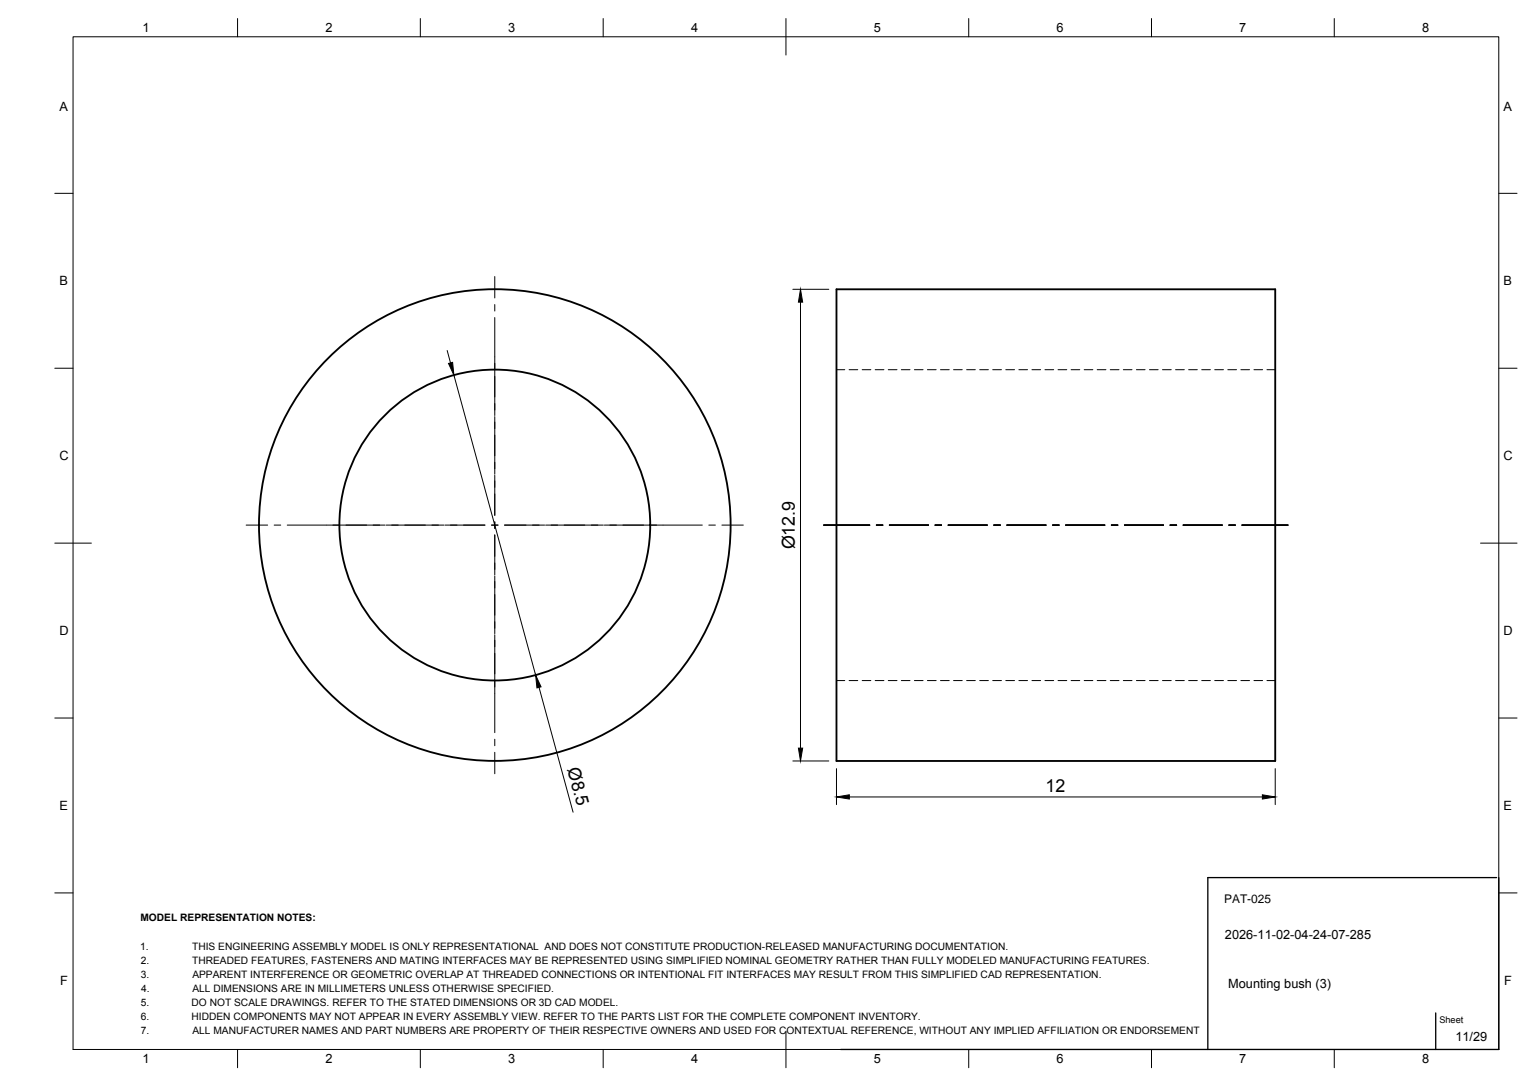
ISO-10303-21;
HEADER;
/* Generated by software containing ST-Developer
 * from STEP Tools, Inc. (www.steptools.com) 
 */

FILE_DESCRIPTION(
/* description */ ('Counter shaft with two pulleys and keyed hub'),
/* implementation_level */ '2;1');

FILE_NAME(
/* name */ 'Mounting bush (3).step',
/* time_stamp */ '2026-10-27T10:46:10-07:00',
/* author */ (''),
/* organization */ (''),
/* preprocessor_version */ 'ST-DEVELOPER v20.2',
/* originating_system */ 'Autodesk Translation Framework v15.17.0.0',
/* authorisation */ '');

FILE_SCHEMA (('AUTOMOTIVE_DESIGN { 1 0 10303 214 3 1 1 }'));
ENDSEC;

DATA;
#10=MECHANICAL_DESIGN_GEOMETRIC_PRESENTATION_REPRESENTATION('',(#296),#10821);
#246=SHAPE_REPRESENTATION_RELATIONSHIP('SRR','None',#10932,#271);
#271=ADVANCED_BREP_SHAPE_REPRESENTATION('',(#322),#10800);
#296=STYLED_ITEM('',(#11128),#322);
#322=MANIFOLD_SOLID_BREP('Body1',#5579);
#354=FACE_BOUND('',#953,.T.);
#355=FACE_BOUND('',#955,.T.);
#455=PLANE('',#5946);
#456=PLANE('',#5947);
#622=FACE_OUTER_BOUND('',#950,.T.);
#623=FACE_OUTER_BOUND('',#951,.T.);
#624=FACE_OUTER_BOUND('',#952,.T.);
#625=FACE_OUTER_BOUND('',#954,.T.);
#950=EDGE_LOOP('',(#3761,#3762,#3763,#3764));
#951=EDGE_LOOP('',(#3765,#3766,#3767,#3768));
#952=EDGE_LOOP('',(#3769));
#953=EDGE_LOOP('',(#3770));
#954=EDGE_LOOP('',(#3771));
#955=EDGE_LOOP('',(#3772));
#1353=LINE('',#8469,#1742);
#1354=LINE('',#8475,#1743);
#1742=VECTOR('',#6735,0.425);
#1743=VECTOR('',#6742,0.645);
#2105=CIRCLE('',#5941,0.425);
#2106=CIRCLE('',#5942,0.425);
#2107=CIRCLE('',#5944,0.645);
#2108=CIRCLE('',#5945,0.645);
#2428=VERTEX_POINT('',#8466);
#2429=VERTEX_POINT('',#8468);
#2430=VERTEX_POINT('',#8472);
#2431=VERTEX_POINT('',#8474);
#2953=EDGE_CURVE('',#2428,#2428,#2105,.T.);
#2954=EDGE_CURVE('',#2428,#2429,#1353,.T.);
#2955=EDGE_CURVE('',#2429,#2429,#2106,.T.);
#2956=EDGE_CURVE('',#2430,#2430,#2107,.T.);
#2957=EDGE_CURVE('',#2430,#2431,#1354,.T.);
#2958=EDGE_CURVE('',#2431,#2431,#2108,.T.);
#3761=ORIENTED_EDGE('',*,*,#2953,.F.);
#3762=ORIENTED_EDGE('',*,*,#2954,.T.);
#3763=ORIENTED_EDGE('',*,*,#2955,.T.);
#3764=ORIENTED_EDGE('',*,*,#2954,.F.);
#3765=ORIENTED_EDGE('',*,*,#2956,.F.);
#3766=ORIENTED_EDGE('',*,*,#2957,.T.);
#3767=ORIENTED_EDGE('',*,*,#2958,.T.);
#3768=ORIENTED_EDGE('',*,*,#2957,.F.);
#3769=ORIENTED_EDGE('',*,*,#2956,.T.);
#3770=ORIENTED_EDGE('',*,*,#2953,.T.);
#3771=ORIENTED_EDGE('',*,*,#2958,.F.);
#3772=ORIENTED_EDGE('',*,*,#2955,.F.);
#5123=CYLINDRICAL_SURFACE('',#5940,0.425);
#5124=CYLINDRICAL_SURFACE('',#5943,0.645);
#5293=ADVANCED_FACE('',(#622),#5123,.F.);
#5294=ADVANCED_FACE('',(#623),#5124,.T.);
#5295=ADVANCED_FACE('',(#624,#354),#455,.T.);
#5296=ADVANCED_FACE('',(#625,#355),#456,.F.);
#5579=CLOSED_SHELL('',(#5293,#5294,#5295,#5296));
#5939=AXIS2_PLACEMENT_3D('',#8464,#6729,#6730);
#5940=AXIS2_PLACEMENT_3D('',#8465,#6731,#6732);
#5941=AXIS2_PLACEMENT_3D('',#8467,#6733,#6734);
#5942=AXIS2_PLACEMENT_3D('',#8470,#6736,#6737);
#5943=AXIS2_PLACEMENT_3D('',#8471,#6738,#6739);
#5944=AXIS2_PLACEMENT_3D('',#8473,#6740,#6741);
#5945=AXIS2_PLACEMENT_3D('',#8476,#6743,#6744);
#5946=AXIS2_PLACEMENT_3D('',#8477,#6745,#6746);
#5947=AXIS2_PLACEMENT_3D('',#8478,#6747,#6748);
#6729=DIRECTION('axis',(0.,0.,1.));
#6730=DIRECTION('refdir',(1.,0.,0.));
#6731=DIRECTION('center_axis',(0.,0.,1.));
#6732=DIRECTION('ref_axis',(1.,0.,0.));
#6733=DIRECTION('center_axis',(0.,0.,-1.));
#6734=DIRECTION('ref_axis',(1.,0.,0.));
#6735=DIRECTION('',(0.,0.,-1.));
#6736=DIRECTION('center_axis',(0.,0.,-1.));
#6737=DIRECTION('ref_axis',(1.,0.,0.));
#6738=DIRECTION('center_axis',(0.,0.,1.));
#6739=DIRECTION('ref_axis',(1.,0.,0.));
#6740=DIRECTION('center_axis',(0.,0.,1.));
#6741=DIRECTION('ref_axis',(1.,0.,0.));
#6742=DIRECTION('',(0.,0.,-1.));
#6743=DIRECTION('center_axis',(0.,0.,1.));
#6744=DIRECTION('ref_axis',(1.,0.,0.));
#6745=DIRECTION('center_axis',(0.,0.,1.));
#6746=DIRECTION('ref_axis',(1.,0.,0.));
#6747=DIRECTION('center_axis',(0.,0.,1.));
#6748=DIRECTION('ref_axis',(1.,0.,0.));
#8464=CARTESIAN_POINT('',(0.,0.,0.));
#8465=CARTESIAN_POINT('Origin',(4.75,20.,1.2));
#8466=CARTESIAN_POINT('',(4.325,20.,2.4));
#8467=CARTESIAN_POINT('Origin',(4.75,20.,2.4));
#8468=CARTESIAN_POINT('',(4.325,20.,1.2));
#8469=CARTESIAN_POINT('',(4.325,20.,1.2));
#8470=CARTESIAN_POINT('Origin',(4.75,20.,1.2));
#8471=CARTESIAN_POINT('Origin',(4.75,20.,1.2));
#8472=CARTESIAN_POINT('',(4.105,20.,2.4));
#8473=CARTESIAN_POINT('Origin',(4.75,20.,2.4));
#8474=CARTESIAN_POINT('',(4.105,20.,1.2));
#8475=CARTESIAN_POINT('',(4.105,20.,1.2));
#8476=CARTESIAN_POINT('Origin',(4.75,20.,1.2));
#8477=CARTESIAN_POINT('Origin',(4.75,20.,2.4));
#8478=CARTESIAN_POINT('Origin',(4.75,20.,1.2));
#10770=UNCERTAINTY_MEASURE_WITH_UNIT(LENGTH_MEASURE(0.001),#10822,
'DISTANCE_ACCURACY_VALUE',
'Maximum model space distance between geometric entities at asserted c
onnectivities');
#10791=UNCERTAINTY_MEASURE_WITH_UNIT(LENGTH_MEASURE(0.001),#10822,
'DISTANCE_ACCURACY_VALUE',
'Maximum model space distance between geometric entities at asserted c
onnectivities');
#10800=(
GEOMETRIC_REPRESENTATION_CONTEXT(3)
GLOBAL_UNCERTAINTY_ASSIGNED_CONTEXT((#10770))
GLOBAL_UNIT_ASSIGNED_CONTEXT((#10822,#10824,#10825))
REPRESENTATION_CONTEXT('','3D')
);
#10821=(
GEOMETRIC_REPRESENTATION_CONTEXT(3)
GLOBAL_UNCERTAINTY_ASSIGNED_CONTEXT((#10791))
GLOBAL_UNIT_ASSIGNED_CONTEXT((#10822,#10824,#10825))
REPRESENTATION_CONTEXT('','3D')
);
#10822=(
LENGTH_UNIT()
NAMED_UNIT(*)
SI_UNIT(.CENTI.,.METRE.)
);
#10824=(
NAMED_UNIT(*)
PLANE_ANGLE_UNIT()
SI_UNIT($,.RADIAN.)
);
#10825=(
NAMED_UNIT(*)
SI_UNIT($,.STERADIAN.)
SOLID_ANGLE_UNIT()
);
#10834=SHAPE_DEFINITION_REPRESENTATION(#10863,#10932);
#10863=PRODUCT_DEFINITION_SHAPE('',$,#10962);
#10932=SHAPE_REPRESENTATION('',(#5939),#10800);
#10953=PRODUCT_DEFINITION_CONTEXT('part definition',#11042,'design');
#10962=PRODUCT_DEFINITION('Mounting bush (3)','Mounting bush (3)',#10991,
#10953);
#10991=PRODUCT_DEFINITION_FORMATION('',$,#11052);
#11042=APPLICATION_CONTEXT(
'Core Data for Automotive Mechanical Design Process');
#11043=PRODUCT_CONTEXT('part definition',#11042,'mechanical');
#11052=PRODUCT('Mounting bush (3)','Mounting bush (3)','Mounting bush (3)',(#11043));
#11122=COLOUR_RGB('Sky Blue',0.24,0.69,0.87);
#11123=FILL_AREA_STYLE_COLOUR('',#11122);
#11124=FILL_AREA_STYLE('',(#11123));
#11125=SURFACE_STYLE_FILL_AREA(#11124);
#11126=SURFACE_SIDE_STYLE('',(#11125));
#11127=SURFACE_STYLE_USAGE(.BOTH.,#11126);
#11128=PRESENTATION_STYLE_ASSIGNMENT((#11127));
ENDSEC;
END-ISO-10303-21;
